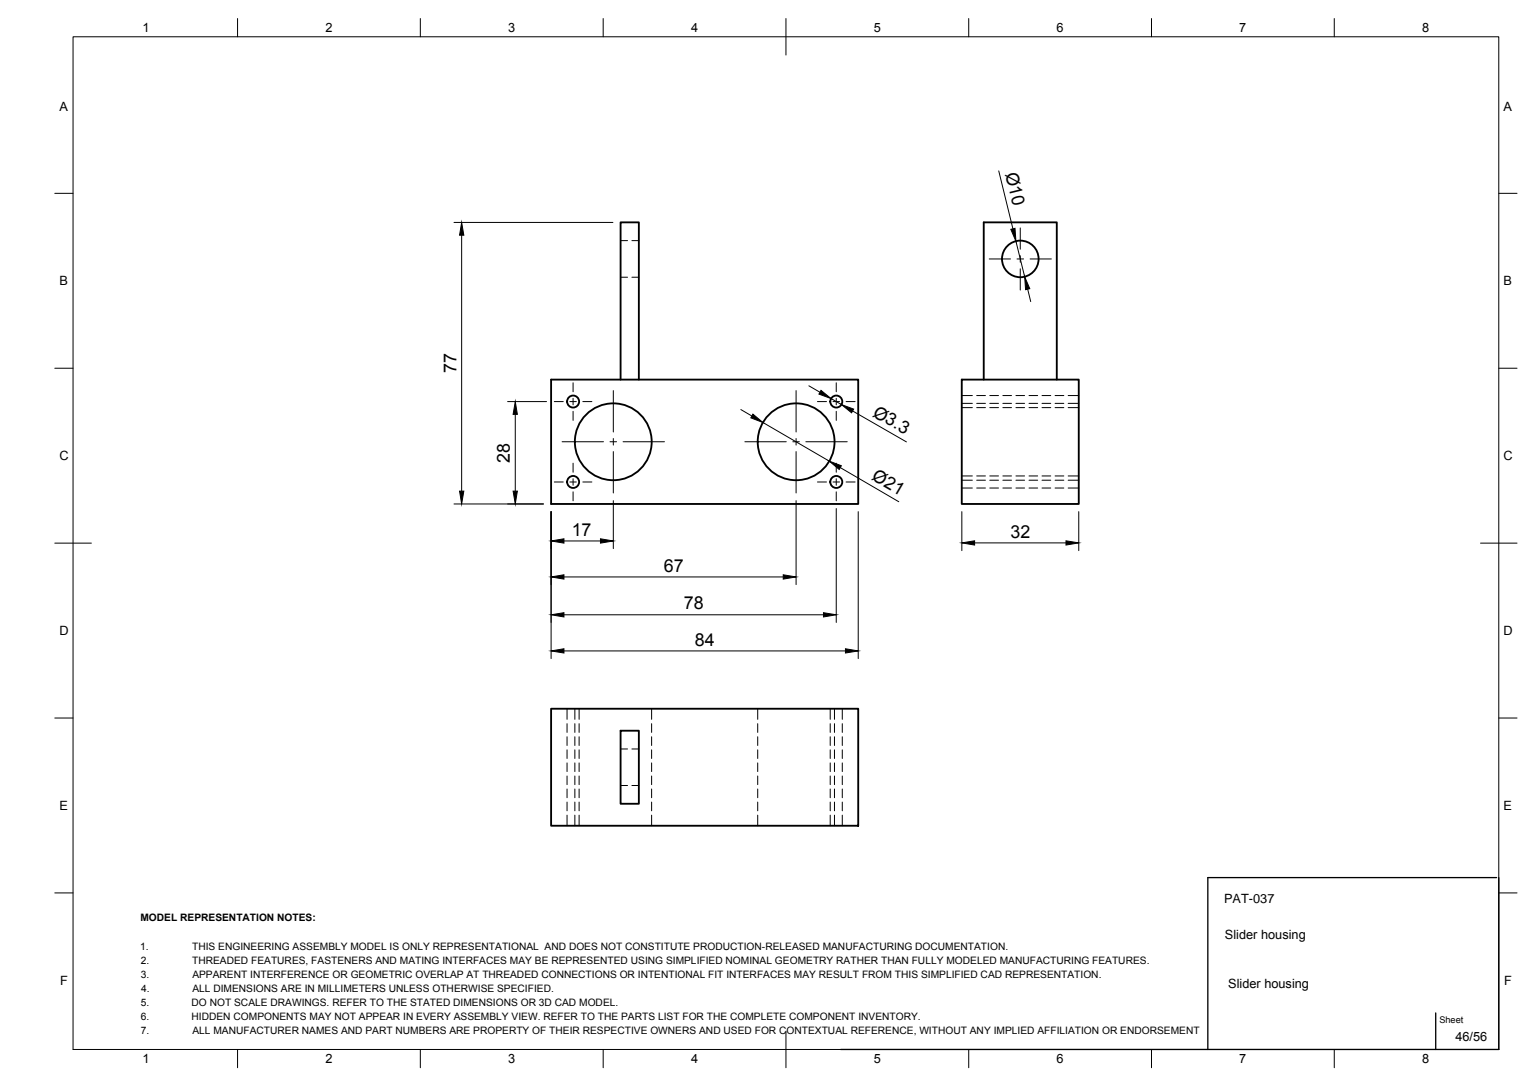
ISO-10303-21;
HEADER;
/* Generated by software containing ST-Developer
 * from STEP Tools, Inc. (www.steptools.com) 
 */

FILE_DESCRIPTION(
/* description */ ('Flywheel Crank-Slider'),
/* implementation_level */ '2;1');

FILE_NAME(
/* name */ 'Slider housing.step',
/* time_stamp */ '2026-10-28T03:23:13-07:00',
/* author */ (''),
/* organization */ (''),
/* preprocessor_version */ 'ST-DEVELOPER v20.2',
/* originating_system */ 'Autodesk Translation Framework v15.17.0.0',
/* authorisation */ '');

FILE_SCHEMA (('AUTOMOTIVE_DESIGN { 1 0 10303 214 3 1 1 }'));
ENDSEC;

DATA;
#10=MECHANICAL_DESIGN_GEOMETRIC_PRESENTATION_REPRESENTATION('',(#719),#17322);
#606=SHAPE_REPRESENTATION_RELATIONSHIP('SRR','None',#17607,#658);
#658=ADVANCED_BREP_SHAPE_REPRESENTATION('',(#776),#17311);
#719=STYLED_ITEM('',(#17910),#776);
#776=MANIFOLD_SOLID_BREP('Body1',#9101);
#952=FACE_BOUND('',#2457,.T.);
#953=FACE_BOUND('',#2462,.T.);
#954=FACE_BOUND('',#2471,.T.);
#955=FACE_BOUND('',#2472,.T.);
#956=FACE_BOUND('',#2473,.T.);
#957=FACE_BOUND('',#2474,.T.);
#958=FACE_BOUND('',#2475,.T.);
#959=FACE_BOUND('',#2476,.T.);
#960=FACE_BOUND('',#2479,.T.);
#961=FACE_BOUND('',#2480,.T.);
#962=FACE_BOUND('',#2481,.T.);
#963=FACE_BOUND('',#2482,.T.);
#964=FACE_BOUND('',#2483,.T.);
#965=FACE_BOUND('',#2484,.T.);
#966=FACE_BOUND('',#2486,.T.);
#1259=PLANE('',#10539);
#1260=PLANE('',#10540);
#1261=PLANE('',#10541);
#1262=PLANE('',#10542);
#1263=PLANE('',#10543);
#1264=PLANE('',#10562);
#1265=PLANE('',#10563);
#1266=PLANE('',#10564);
#1267=PLANE('',#10565);
#1268=PLANE('',#10566);
#1269=PLANE('',#10567);
#1753=FACE_OUTER_BOUND('',#2455,.T.);
#1754=FACE_OUTER_BOUND('',#2456,.T.);
#1755=FACE_OUTER_BOUND('',#2458,.T.);
#1756=FACE_OUTER_BOUND('',#2459,.T.);
#1757=FACE_OUTER_BOUND('',#2460,.T.);
#1758=FACE_OUTER_BOUND('',#2461,.T.);
#1759=FACE_OUTER_BOUND('',#2463,.T.);
#1760=FACE_OUTER_BOUND('',#2464,.T.);
#1761=FACE_OUTER_BOUND('',#2465,.T.);
#1762=FACE_OUTER_BOUND('',#2466,.T.);
#1763=FACE_OUTER_BOUND('',#2467,.T.);
#1764=FACE_OUTER_BOUND('',#2468,.T.);
#1765=FACE_OUTER_BOUND('',#2469,.T.);
#1766=FACE_OUTER_BOUND('',#2470,.T.);
#1767=FACE_OUTER_BOUND('',#2477,.T.);
#1768=FACE_OUTER_BOUND('',#2478,.T.);
#1769=FACE_OUTER_BOUND('',#2485,.T.);
#1770=FACE_OUTER_BOUND('',#2487,.T.);
#2455=EDGE_LOOP('',(#7910,#7911,#7912,#7913));
#2456=EDGE_LOOP('',(#7914,#7915,#7916,#7917));
#2457=EDGE_LOOP('',(#7918));
#2458=EDGE_LOOP('',(#7919,#7920,#7921,#7922));
#2459=EDGE_LOOP('',(#7923,#7924,#7925,#7926));
#2460=EDGE_LOOP('',(#7927,#7928,#7929,#7930));
#2461=EDGE_LOOP('',(#7931,#7932,#7933,#7934));
#2462=EDGE_LOOP('',(#7935));
#2463=EDGE_LOOP('',(#7936,#7937,#7938,#7939));
#2464=EDGE_LOOP('',(#7940,#7941,#7942,#7943));
#2465=EDGE_LOOP('',(#7944,#7945,#7946,#7947));
#2466=EDGE_LOOP('',(#7948,#7949,#7950,#7951));
#2467=EDGE_LOOP('',(#7952,#7953,#7954,#7955));
#2468=EDGE_LOOP('',(#7956,#7957,#7958,#7959));
#2469=EDGE_LOOP('',(#7960,#7961,#7962,#7963));
#2470=EDGE_LOOP('',(#7964,#7965,#7966,#7967));
#2471=EDGE_LOOP('',(#7968));
#2472=EDGE_LOOP('',(#7969));
#2473=EDGE_LOOP('',(#7970));
#2474=EDGE_LOOP('',(#7971));
#2475=EDGE_LOOP('',(#7972));
#2476=EDGE_LOOP('',(#7973));
#2477=EDGE_LOOP('',(#7974,#7975,#7976,#7977));
#2478=EDGE_LOOP('',(#7978,#7979,#7980,#7981));
#2479=EDGE_LOOP('',(#7982));
#2480=EDGE_LOOP('',(#7983));
#2481=EDGE_LOOP('',(#7984));
#2482=EDGE_LOOP('',(#7985));
#2483=EDGE_LOOP('',(#7986));
#2484=EDGE_LOOP('',(#7987));
#2485=EDGE_LOOP('',(#7988,#7989,#7990,#7991));
#2486=EDGE_LOOP('',(#7992,#7993,#7994,#7995));
#2487=EDGE_LOOP('',(#7996,#7997,#7998,#7999));
#3102=LINE('',#16647,#3713);
#3103=LINE('',#16652,#3714);
#3104=LINE('',#16654,#3715);
#3105=LINE('',#16656,#3716);
#3106=LINE('',#16657,#3717);
#3107=LINE('',#16660,#3718);
#3108=LINE('',#16662,#3719);
#3109=LINE('',#16663,#3720);
#3110=LINE('',#16666,#3721);
#3111=LINE('',#16668,#3722);
#3112=LINE('',#16669,#3723);
#3113=LINE('',#16671,#3724);
#3114=LINE('',#16673,#3725);
#3115=LINE('',#16678,#3726);
#3116=LINE('',#16684,#3727);
#3117=LINE('',#16690,#3728);
#3118=LINE('',#16696,#3729);
#3119=LINE('',#16702,#3730);
#3120=LINE('',#16708,#3731);
#3121=LINE('',#16713,#3732);
#3122=LINE('',#16715,#3733);
#3123=LINE('',#16717,#3734);
#3124=LINE('',#16718,#3735);
#3125=LINE('',#16721,#3736);
#3126=LINE('',#16723,#3737);
#3127=LINE('',#16724,#3738);
#3128=LINE('',#16727,#3739);
#3129=LINE('',#16729,#3740);
#3130=LINE('',#16730,#3741);
#3131=LINE('',#16732,#3742);
#3132=LINE('',#16733,#3743);
#3713=VECTOR('',#13022,0.5);
#3714=VECTOR('',#13027,1.);
#3715=VECTOR('',#13028,1.);
#3716=VECTOR('',#13029,1.);
#3717=VECTOR('',#13030,1.);
#3718=VECTOR('',#13033,1.);
#3719=VECTOR('',#13034,1.);
#3720=VECTOR('',#13035,1.);
#3721=VECTOR('',#13038,1.);
#3722=VECTOR('',#13039,1.);
#3723=VECTOR('',#13040,1.);
#3724=VECTOR('',#13043,1.);
#3725=VECTOR('',#13046,1.);
#3726=VECTOR('',#13051,0.165);
#3727=VECTOR('',#13058,0.165);
#3728=VECTOR('',#13065,0.165);
#3729=VECTOR('',#13072,0.165);
#3730=VECTOR('',#13079,1.05);
#3731=VECTOR('',#13086,1.05);
#3732=VECTOR('',#13091,1.);
#3733=VECTOR('',#13092,1.);
#3734=VECTOR('',#13093,1.);
#3735=VECTOR('',#13094,1.);
#3736=VECTOR('',#13097,1.);
#3737=VECTOR('',#13098,1.);
#3738=VECTOR('',#13099,1.);
#3739=VECTOR('',#13102,1.);
#3740=VECTOR('',#13103,1.);
#3741=VECTOR('',#13104,1.);
#3742=VECTOR('',#13107,1.);
#3743=VECTOR('',#13108,1.);
#4192=CIRCLE('',#10537,0.5);
#4193=CIRCLE('',#10538,0.5);
#4194=CIRCLE('',#10545,0.165);
#4195=CIRCLE('',#10546,0.165);
#4196=CIRCLE('',#10548,0.165);
#4197=CIRCLE('',#10549,0.165);
#4198=CIRCLE('',#10551,0.165);
#4199=CIRCLE('',#10552,0.165);
#4200=CIRCLE('',#10554,0.165);
#4201=CIRCLE('',#10555,0.165);
#4202=CIRCLE('',#10557,1.05);
#4203=CIRCLE('',#10558,1.05);
#4204=CIRCLE('',#10560,1.05);
#4205=CIRCLE('',#10561,1.05);
#4879=VERTEX_POINT('',#16644);
#4880=VERTEX_POINT('',#16646);
#4881=VERTEX_POINT('',#16650);
#4882=VERTEX_POINT('',#16651);
#4883=VERTEX_POINT('',#16653);
#4884=VERTEX_POINT('',#16655);
#4885=VERTEX_POINT('',#16659);
#4886=VERTEX_POINT('',#16661);
#4887=VERTEX_POINT('',#16665);
#4888=VERTEX_POINT('',#16667);
#4889=VERTEX_POINT('',#16675);
#4890=VERTEX_POINT('',#16677);
#4891=VERTEX_POINT('',#16681);
#4892=VERTEX_POINT('',#16683);
#4893=VERTEX_POINT('',#16687);
#4894=VERTEX_POINT('',#16689);
#4895=VERTEX_POINT('',#16693);
#4896=VERTEX_POINT('',#16695);
#4897=VERTEX_POINT('',#16699);
#4898=VERTEX_POINT('',#16701);
#4899=VERTEX_POINT('',#16705);
#4900=VERTEX_POINT('',#16707);
#4901=VERTEX_POINT('',#16711);
#4902=VERTEX_POINT('',#16712);
#4903=VERTEX_POINT('',#16714);
#4904=VERTEX_POINT('',#16716);
#4905=VERTEX_POINT('',#16720);
#4906=VERTEX_POINT('',#16722);
#4907=VERTEX_POINT('',#16726);
#4908=VERTEX_POINT('',#16728);
#5912=EDGE_CURVE('',#4879,#4879,#4192,.T.);
#5913=EDGE_CURVE('',#4879,#4880,#3102,.T.);
#5914=EDGE_CURVE('',#4880,#4880,#4193,.T.);
#5915=EDGE_CURVE('',#4881,#4882,#3103,.T.);
#5916=EDGE_CURVE('',#4881,#4883,#3104,.T.);
#5917=EDGE_CURVE('',#4883,#4884,#3105,.T.);
#5918=EDGE_CURVE('',#4884,#4882,#3106,.T.);
#5919=EDGE_CURVE('',#4885,#4881,#3107,.T.);
#5920=EDGE_CURVE('',#4886,#4885,#3108,.T.);
#5921=EDGE_CURVE('',#4883,#4886,#3109,.T.);
#5922=EDGE_CURVE('',#4882,#4887,#3110,.T.);
#5923=EDGE_CURVE('',#4884,#4888,#3111,.T.);
#5924=EDGE_CURVE('',#4887,#4888,#3112,.T.);
#5925=EDGE_CURVE('',#4888,#4886,#3113,.T.);
#5926=EDGE_CURVE('',#4887,#4885,#3114,.T.);
#5927=EDGE_CURVE('',#4889,#4889,#4194,.T.);
#5928=EDGE_CURVE('',#4889,#4890,#3115,.T.);
#5929=EDGE_CURVE('',#4890,#4890,#4195,.T.);
#5930=EDGE_CURVE('',#4891,#4891,#4196,.T.);
#5931=EDGE_CURVE('',#4891,#4892,#3116,.T.);
#5932=EDGE_CURVE('',#4892,#4892,#4197,.T.);
#5933=EDGE_CURVE('',#4893,#4893,#4198,.T.);
#5934=EDGE_CURVE('',#4893,#4894,#3117,.T.);
#5935=EDGE_CURVE('',#4894,#4894,#4199,.T.);
#5936=EDGE_CURVE('',#4895,#4895,#4200,.T.);
#5937=EDGE_CURVE('',#4895,#4896,#3118,.T.);
#5938=EDGE_CURVE('',#4896,#4896,#4201,.T.);
#5939=EDGE_CURVE('',#4897,#4897,#4202,.T.);
#5940=EDGE_CURVE('',#4897,#4898,#3119,.T.);
#5941=EDGE_CURVE('',#4898,#4898,#4203,.T.);
#5942=EDGE_CURVE('',#4899,#4899,#4204,.T.);
#5943=EDGE_CURVE('',#4899,#4900,#3120,.T.);
#5944=EDGE_CURVE('',#4900,#4900,#4205,.T.);
#5945=EDGE_CURVE('',#4901,#4902,#3121,.T.);
#5946=EDGE_CURVE('',#4902,#4903,#3122,.T.);
#5947=EDGE_CURVE('',#4904,#4903,#3123,.T.);
#5948=EDGE_CURVE('',#4901,#4904,#3124,.T.);
#5949=EDGE_CURVE('',#4905,#4901,#3125,.T.);
#5950=EDGE_CURVE('',#4906,#4904,#3126,.T.);
#5951=EDGE_CURVE('',#4905,#4906,#3127,.T.);
#5952=EDGE_CURVE('',#4907,#4905,#3128,.T.);
#5953=EDGE_CURVE('',#4908,#4906,#3129,.T.);
#5954=EDGE_CURVE('',#4907,#4908,#3130,.T.);
#5955=EDGE_CURVE('',#4902,#4907,#3131,.T.);
#5956=EDGE_CURVE('',#4903,#4908,#3132,.T.);
#7910=ORIENTED_EDGE('',*,*,#5912,.F.);
#7911=ORIENTED_EDGE('',*,*,#5913,.T.);
#7912=ORIENTED_EDGE('',*,*,#5914,.F.);
#7913=ORIENTED_EDGE('',*,*,#5913,.F.);
#7914=ORIENTED_EDGE('',*,*,#5915,.F.);
#7915=ORIENTED_EDGE('',*,*,#5916,.T.);
#7916=ORIENTED_EDGE('',*,*,#5917,.T.);
#7917=ORIENTED_EDGE('',*,*,#5918,.T.);
#7918=ORIENTED_EDGE('',*,*,#5912,.T.);
#7919=ORIENTED_EDGE('',*,*,#5919,.F.);
#7920=ORIENTED_EDGE('',*,*,#5920,.F.);
#7921=ORIENTED_EDGE('',*,*,#5921,.F.);
#7922=ORIENTED_EDGE('',*,*,#5916,.F.);
#7923=ORIENTED_EDGE('',*,*,#5922,.F.);
#7924=ORIENTED_EDGE('',*,*,#5918,.F.);
#7925=ORIENTED_EDGE('',*,*,#5923,.T.);
#7926=ORIENTED_EDGE('',*,*,#5924,.F.);
#7927=ORIENTED_EDGE('',*,*,#5917,.F.);
#7928=ORIENTED_EDGE('',*,*,#5921,.T.);
#7929=ORIENTED_EDGE('',*,*,#5925,.F.);
#7930=ORIENTED_EDGE('',*,*,#5923,.F.);
#7931=ORIENTED_EDGE('',*,*,#5926,.F.);
#7932=ORIENTED_EDGE('',*,*,#5924,.T.);
#7933=ORIENTED_EDGE('',*,*,#5925,.T.);
#7934=ORIENTED_EDGE('',*,*,#5920,.T.);
#7935=ORIENTED_EDGE('',*,*,#5914,.T.);
#7936=ORIENTED_EDGE('',*,*,#5927,.F.);
#7937=ORIENTED_EDGE('',*,*,#5928,.T.);
#7938=ORIENTED_EDGE('',*,*,#5929,.F.);
#7939=ORIENTED_EDGE('',*,*,#5928,.F.);
#7940=ORIENTED_EDGE('',*,*,#5930,.F.);
#7941=ORIENTED_EDGE('',*,*,#5931,.T.);
#7942=ORIENTED_EDGE('',*,*,#5932,.F.);
#7943=ORIENTED_EDGE('',*,*,#5931,.F.);
#7944=ORIENTED_EDGE('',*,*,#5933,.F.);
#7945=ORIENTED_EDGE('',*,*,#5934,.T.);
#7946=ORIENTED_EDGE('',*,*,#5935,.F.);
#7947=ORIENTED_EDGE('',*,*,#5934,.F.);
#7948=ORIENTED_EDGE('',*,*,#5936,.F.);
#7949=ORIENTED_EDGE('',*,*,#5937,.T.);
#7950=ORIENTED_EDGE('',*,*,#5938,.F.);
#7951=ORIENTED_EDGE('',*,*,#5937,.F.);
#7952=ORIENTED_EDGE('',*,*,#5939,.F.);
#7953=ORIENTED_EDGE('',*,*,#5940,.T.);
#7954=ORIENTED_EDGE('',*,*,#5941,.F.);
#7955=ORIENTED_EDGE('',*,*,#5940,.F.);
#7956=ORIENTED_EDGE('',*,*,#5942,.F.);
#7957=ORIENTED_EDGE('',*,*,#5943,.T.);
#7958=ORIENTED_EDGE('',*,*,#5944,.F.);
#7959=ORIENTED_EDGE('',*,*,#5943,.F.);
#7960=ORIENTED_EDGE('',*,*,#5945,.T.);
#7961=ORIENTED_EDGE('',*,*,#5946,.T.);
#7962=ORIENTED_EDGE('',*,*,#5947,.F.);
#7963=ORIENTED_EDGE('',*,*,#5948,.F.);
#7964=ORIENTED_EDGE('',*,*,#5949,.T.);
#7965=ORIENTED_EDGE('',*,*,#5948,.T.);
#7966=ORIENTED_EDGE('',*,*,#5950,.F.);
#7967=ORIENTED_EDGE('',*,*,#5951,.F.);
#7968=ORIENTED_EDGE('',*,*,#5944,.T.);
#7969=ORIENTED_EDGE('',*,*,#5941,.T.);
#7970=ORIENTED_EDGE('',*,*,#5938,.T.);
#7971=ORIENTED_EDGE('',*,*,#5935,.T.);
#7972=ORIENTED_EDGE('',*,*,#5932,.T.);
#7973=ORIENTED_EDGE('',*,*,#5929,.T.);
#7974=ORIENTED_EDGE('',*,*,#5952,.T.);
#7975=ORIENTED_EDGE('',*,*,#5951,.T.);
#7976=ORIENTED_EDGE('',*,*,#5953,.F.);
#7977=ORIENTED_EDGE('',*,*,#5954,.F.);
#7978=ORIENTED_EDGE('',*,*,#5955,.T.);
#7979=ORIENTED_EDGE('',*,*,#5954,.T.);
#7980=ORIENTED_EDGE('',*,*,#5956,.F.);
#7981=ORIENTED_EDGE('',*,*,#5946,.F.);
#7982=ORIENTED_EDGE('',*,*,#5942,.T.);
#7983=ORIENTED_EDGE('',*,*,#5939,.T.);
#7984=ORIENTED_EDGE('',*,*,#5936,.T.);
#7985=ORIENTED_EDGE('',*,*,#5933,.T.);
#7986=ORIENTED_EDGE('',*,*,#5930,.T.);
#7987=ORIENTED_EDGE('',*,*,#5927,.T.);
#7988=ORIENTED_EDGE('',*,*,#5956,.T.);
#7989=ORIENTED_EDGE('',*,*,#5953,.T.);
#7990=ORIENTED_EDGE('',*,*,#5950,.T.);
#7991=ORIENTED_EDGE('',*,*,#5947,.T.);
#7992=ORIENTED_EDGE('',*,*,#5919,.T.);
#7993=ORIENTED_EDGE('',*,*,#5915,.T.);
#7994=ORIENTED_EDGE('',*,*,#5922,.T.);
#7995=ORIENTED_EDGE('',*,*,#5926,.T.);
#7996=ORIENTED_EDGE('',*,*,#5955,.F.);
#7997=ORIENTED_EDGE('',*,*,#5945,.F.);
#7998=ORIENTED_EDGE('',*,*,#5949,.F.);
#7999=ORIENTED_EDGE('',*,*,#5952,.F.);
#8473=CYLINDRICAL_SURFACE('',#10536,0.5);
#8474=CYLINDRICAL_SURFACE('',#10544,0.165);
#8475=CYLINDRICAL_SURFACE('',#10547,0.165);
#8476=CYLINDRICAL_SURFACE('',#10550,0.165);
#8477=CYLINDRICAL_SURFACE('',#10553,0.165);
#8478=CYLINDRICAL_SURFACE('',#10556,1.05);
#8479=CYLINDRICAL_SURFACE('',#10559,1.05);
#8944=ADVANCED_FACE('',(#1753),#8473,.F.);
#8945=ADVANCED_FACE('',(#1754,#952),#1259,.F.);
#8946=ADVANCED_FACE('',(#1755),#1260,.T.);
#8947=ADVANCED_FACE('',(#1756),#1261,.T.);
#8948=ADVANCED_FACE('',(#1757),#1262,.T.);
#8949=ADVANCED_FACE('',(#1758,#953),#1263,.T.);
#8950=ADVANCED_FACE('',(#1759),#8474,.F.);
#8951=ADVANCED_FACE('',(#1760),#8475,.F.);
#8952=ADVANCED_FACE('',(#1761),#8476,.F.);
#8953=ADVANCED_FACE('',(#1762),#8477,.F.);
#8954=ADVANCED_FACE('',(#1763),#8478,.F.);
#8955=ADVANCED_FACE('',(#1764),#8479,.F.);
#8956=ADVANCED_FACE('',(#1765),#1264,.T.);
#8957=ADVANCED_FACE('',(#1766,#954,#955,#956,#957,#958,#959),#1265,.T.);
#8958=ADVANCED_FACE('',(#1767),#1266,.T.);
#8959=ADVANCED_FACE('',(#1768,#960,#961,#962,#963,#964,#965),#1267,.T.);
#8960=ADVANCED_FACE('',(#1769,#966),#1268,.T.);
#8961=ADVANCED_FACE('',(#1770),#1269,.F.);
#9101=CLOSED_SHELL('',(#8944,#8945,#8946,#8947,#8948,#8949,#8950,#8951,
#8952,#8953,#8954,#8955,#8956,#8957,#8958,#8959,#8960,#8961));
#10535=AXIS2_PLACEMENT_3D('',#16642,#13016,#13017);
#10536=AXIS2_PLACEMENT_3D('',#16643,#13018,#13019);
#10537=AXIS2_PLACEMENT_3D('',#16645,#13020,#13021);
#10538=AXIS2_PLACEMENT_3D('',#16648,#13023,#13024);
#10539=AXIS2_PLACEMENT_3D('',#16649,#13025,#13026);
#10540=AXIS2_PLACEMENT_3D('',#16658,#13031,#13032);
#10541=AXIS2_PLACEMENT_3D('',#16664,#13036,#13037);
#10542=AXIS2_PLACEMENT_3D('',#16670,#13041,#13042);
#10543=AXIS2_PLACEMENT_3D('',#16672,#13044,#13045);
#10544=AXIS2_PLACEMENT_3D('',#16674,#13047,#13048);
#10545=AXIS2_PLACEMENT_3D('',#16676,#13049,#13050);
#10546=AXIS2_PLACEMENT_3D('',#16679,#13052,#13053);
#10547=AXIS2_PLACEMENT_3D('',#16680,#13054,#13055);
#10548=AXIS2_PLACEMENT_3D('',#16682,#13056,#13057);
#10549=AXIS2_PLACEMENT_3D('',#16685,#13059,#13060);
#10550=AXIS2_PLACEMENT_3D('',#16686,#13061,#13062);
#10551=AXIS2_PLACEMENT_3D('',#16688,#13063,#13064);
#10552=AXIS2_PLACEMENT_3D('',#16691,#13066,#13067);
#10553=AXIS2_PLACEMENT_3D('',#16692,#13068,#13069);
#10554=AXIS2_PLACEMENT_3D('',#16694,#13070,#13071);
#10555=AXIS2_PLACEMENT_3D('',#16697,#13073,#13074);
#10556=AXIS2_PLACEMENT_3D('',#16698,#13075,#13076);
#10557=AXIS2_PLACEMENT_3D('',#16700,#13077,#13078);
#10558=AXIS2_PLACEMENT_3D('',#16703,#13080,#13081);
#10559=AXIS2_PLACEMENT_3D('',#16704,#13082,#13083);
#10560=AXIS2_PLACEMENT_3D('',#16706,#13084,#13085);
#10561=AXIS2_PLACEMENT_3D('',#16709,#13087,#13088);
#10562=AXIS2_PLACEMENT_3D('',#16710,#13089,#13090);
#10563=AXIS2_PLACEMENT_3D('',#16719,#13095,#13096);
#10564=AXIS2_PLACEMENT_3D('',#16725,#13100,#13101);
#10565=AXIS2_PLACEMENT_3D('',#16731,#13105,#13106);
#10566=AXIS2_PLACEMENT_3D('',#16734,#13109,#13110);
#10567=AXIS2_PLACEMENT_3D('',#16735,#13111,#13112);
#13016=DIRECTION('axis',(0.,0.,1.));
#13017=DIRECTION('refdir',(1.,0.,0.));
#13018=DIRECTION('center_axis',(0.,1.,0.));
#13019=DIRECTION('ref_axis',(1.,0.,0.));
#13020=DIRECTION('center_axis',(0.,1.,0.));
#13021=DIRECTION('ref_axis',(1.,0.,0.));
#13022=DIRECTION('',(0.,1.,0.));
#13023=DIRECTION('center_axis',(0.,-1.,0.));
#13024=DIRECTION('ref_axis',(1.,0.,0.));
#13025=DIRECTION('center_axis',(0.,1.,0.));
#13026=DIRECTION('ref_axis',(1.,0.,0.));
#13027=DIRECTION('',(-1.,0.,0.));
#13028=DIRECTION('',(0.,0.,1.));
#13029=DIRECTION('',(-1.,0.,0.));
#13030=DIRECTION('',(0.,0.,-1.));
#13031=DIRECTION('center_axis',(1.,0.,0.));
#13032=DIRECTION('ref_axis',(0.,0.,-1.));
#13033=DIRECTION('',(0.,-1.,0.));
#13034=DIRECTION('',(0.,0.,-1.));
#13035=DIRECTION('',(0.,1.,0.));
#13036=DIRECTION('center_axis',(-1.,0.,0.));
#13037=DIRECTION('ref_axis',(0.,0.,1.));
#13038=DIRECTION('',(0.,1.,0.));
#13039=DIRECTION('',(0.,1.,0.));
#13040=DIRECTION('',(0.,0.,1.));
#13041=DIRECTION('center_axis',(0.,0.,1.));
#13042=DIRECTION('ref_axis',(1.,0.,0.));
#13043=DIRECTION('',(1.,0.,0.));
#13044=DIRECTION('center_axis',(0.,1.,0.));
#13045=DIRECTION('ref_axis',(0.,0.,1.));
#13046=DIRECTION('',(1.,0.,0.));
#13047=DIRECTION('center_axis',(1.,0.,0.));
#13048=DIRECTION('ref_axis',(0.,0.,-1.));
#13049=DIRECTION('center_axis',(1.,0.,0.));
#13050=DIRECTION('ref_axis',(0.,0.,-1.));
#13051=DIRECTION('',(1.,0.,0.));
#13052=DIRECTION('center_axis',(-1.,0.,0.));
#13053=DIRECTION('ref_axis',(0.,0.,-1.));
#13054=DIRECTION('center_axis',(1.,0.,0.));
#13055=DIRECTION('ref_axis',(0.,0.,-1.));
#13056=DIRECTION('center_axis',(1.,0.,0.));
#13057=DIRECTION('ref_axis',(0.,0.,-1.));
#13058=DIRECTION('',(1.,0.,0.));
#13059=DIRECTION('center_axis',(-1.,0.,0.));
#13060=DIRECTION('ref_axis',(0.,0.,-1.));
#13061=DIRECTION('center_axis',(1.,0.,0.));
#13062=DIRECTION('ref_axis',(0.,0.,-1.));
#13063=DIRECTION('center_axis',(1.,0.,0.));
#13064=DIRECTION('ref_axis',(0.,0.,-1.));
#13065=DIRECTION('',(1.,0.,0.));
#13066=DIRECTION('center_axis',(-1.,0.,0.));
#13067=DIRECTION('ref_axis',(0.,0.,-1.));
#13068=DIRECTION('center_axis',(1.,0.,0.));
#13069=DIRECTION('ref_axis',(0.,0.,-1.));
#13070=DIRECTION('center_axis',(1.,0.,0.));
#13071=DIRECTION('ref_axis',(0.,0.,-1.));
#13072=DIRECTION('',(1.,0.,0.));
#13073=DIRECTION('center_axis',(-1.,0.,0.));
#13074=DIRECTION('ref_axis',(0.,0.,-1.));
#13075=DIRECTION('center_axis',(1.,0.,0.));
#13076=DIRECTION('ref_axis',(0.,0.,-1.));
#13077=DIRECTION('center_axis',(1.,0.,0.));
#13078=DIRECTION('ref_axis',(0.,0.,-1.));
#13079=DIRECTION('',(1.,0.,0.));
#13080=DIRECTION('center_axis',(-1.,0.,0.));
#13081=DIRECTION('ref_axis',(0.,0.,-1.));
#13082=DIRECTION('center_axis',(1.,0.,0.));
#13083=DIRECTION('ref_axis',(0.,0.,-1.));
#13084=DIRECTION('center_axis',(1.,0.,0.));
#13085=DIRECTION('ref_axis',(0.,0.,-1.));
#13086=DIRECTION('',(1.,0.,0.));
#13087=DIRECTION('center_axis',(-1.,0.,0.));
#13088=DIRECTION('ref_axis',(0.,0.,-1.));
#13089=DIRECTION('center_axis',(0.,1.,0.));
#13090=DIRECTION('ref_axis',(-1.,0.,0.));
#13091=DIRECTION('',(-1.,0.,0.));
#13092=DIRECTION('',(0.,0.,1.));
#13093=DIRECTION('',(-1.,0.,0.));
#13094=DIRECTION('',(0.,0.,1.));
#13095=DIRECTION('center_axis',(1.,0.,0.));
#13096=DIRECTION('ref_axis',(0.,1.,0.));
#13097=DIRECTION('',(0.,1.,0.));
#13098=DIRECTION('',(0.,1.,0.));
#13099=DIRECTION('',(0.,0.,1.));
#13100=DIRECTION('center_axis',(0.,-1.,0.));
#13101=DIRECTION('ref_axis',(1.,0.,0.));
#13102=DIRECTION('',(1.,0.,0.));
#13103=DIRECTION('',(1.,0.,0.));
#13104=DIRECTION('',(0.,0.,1.));
#13105=DIRECTION('center_axis',(-1.,0.,0.));
#13106=DIRECTION('ref_axis',(0.,-1.,0.));
#13107=DIRECTION('',(0.,-1.,0.));
#13108=DIRECTION('',(0.,-1.,0.));
#13109=DIRECTION('center_axis',(0.,0.,1.));
#13110=DIRECTION('ref_axis',(1.,0.,0.));
#13111=DIRECTION('center_axis',(0.,0.,1.));
#13112=DIRECTION('ref_axis',(1.,0.,0.));
#16642=CARTESIAN_POINT('',(0.,0.,0.));
#16643=CARTESIAN_POINT('Origin',(12.,1.7,10.));
#16644=CARTESIAN_POINT('',(11.5,1.8,10.));
#16645=CARTESIAN_POINT('Origin',(12.,1.8,10.));
#16646=CARTESIAN_POINT('',(11.5,2.3,10.));
#16647=CARTESIAN_POINT('',(11.5,1.7,10.));
#16648=CARTESIAN_POINT('Origin',(12.,2.3,10.));
#16649=CARTESIAN_POINT('Origin',(12.,1.8,8.75));
#16650=CARTESIAN_POINT('',(13.,1.8,6.7));
#16651=CARTESIAN_POINT('',(11.,1.8,6.7));
#16652=CARTESIAN_POINT('',(12.,1.8,6.7));
#16653=CARTESIAN_POINT('',(13.,1.8,11.));
#16654=CARTESIAN_POINT('',(13.,1.8,6.5));
#16655=CARTESIAN_POINT('',(11.,1.8,11.));
#16656=CARTESIAN_POINT('',(13.,1.8,11.));
#16657=CARTESIAN_POINT('',(11.,1.8,11.));
#16658=CARTESIAN_POINT('Origin',(13.,1.8,11.));
#16659=CARTESIAN_POINT('',(13.,2.3,6.7));
#16660=CARTESIAN_POINT('',(13.,0.9,6.7));
#16661=CARTESIAN_POINT('',(13.,2.3,11.));
#16662=CARTESIAN_POINT('',(13.,2.3,6.5));
#16663=CARTESIAN_POINT('',(13.,1.8,11.));
#16664=CARTESIAN_POINT('Origin',(11.,1.8,6.5));
#16665=CARTESIAN_POINT('',(11.,2.3,6.7));
#16666=CARTESIAN_POINT('',(11.,0.9,6.7));
#16667=CARTESIAN_POINT('',(11.,2.3,11.));
#16668=CARTESIAN_POINT('',(11.,1.8,11.));
#16669=CARTESIAN_POINT('',(11.,2.3,11.));
#16670=CARTESIAN_POINT('Origin',(11.,1.8,11.));
#16671=CARTESIAN_POINT('',(13.,2.3,11.));
#16672=CARTESIAN_POINT('Origin',(12.,2.3,8.75));
#16673=CARTESIAN_POINT('',(12.,2.3,6.7));
#16674=CARTESIAN_POINT('Origin',(10.3,3.6,3.9));
#16675=CARTESIAN_POINT('',(10.4,3.6,4.065));
#16676=CARTESIAN_POINT('Origin',(10.4,3.6,3.9));
#16677=CARTESIAN_POINT('',(13.6,3.6,4.065));
#16678=CARTESIAN_POINT('',(10.3,3.6,4.065));
#16679=CARTESIAN_POINT('Origin',(13.6,3.6,3.9));
#16680=CARTESIAN_POINT('Origin',(10.3,-3.6,6.1));
#16681=CARTESIAN_POINT('',(10.4,-3.6,6.265));
#16682=CARTESIAN_POINT('Origin',(10.4,-3.6,6.1));
#16683=CARTESIAN_POINT('',(13.6,-3.6,6.265));
#16684=CARTESIAN_POINT('',(10.3,-3.6,6.265));
#16685=CARTESIAN_POINT('Origin',(13.6,-3.6,6.1));
#16686=CARTESIAN_POINT('Origin',(10.3,-3.6,3.9));
#16687=CARTESIAN_POINT('',(10.4,-3.6,4.065));
#16688=CARTESIAN_POINT('Origin',(10.4,-3.6,3.9));
#16689=CARTESIAN_POINT('',(13.6,-3.6,4.065));
#16690=CARTESIAN_POINT('',(10.3,-3.6,4.065));
#16691=CARTESIAN_POINT('Origin',(13.6,-3.6,3.9));
#16692=CARTESIAN_POINT('Origin',(10.3,3.6,6.1));
#16693=CARTESIAN_POINT('',(10.4,3.6,6.265));
#16694=CARTESIAN_POINT('Origin',(10.4,3.6,6.1));
#16695=CARTESIAN_POINT('',(13.6,3.6,6.265));
#16696=CARTESIAN_POINT('',(10.3,3.6,6.265));
#16697=CARTESIAN_POINT('Origin',(13.6,3.6,6.1));
#16698=CARTESIAN_POINT('Origin',(10.3,-2.5,5.));
#16699=CARTESIAN_POINT('',(10.4,-2.5,6.05));
#16700=CARTESIAN_POINT('Origin',(10.4,-2.5,5.));
#16701=CARTESIAN_POINT('',(13.6,-2.5,6.05));
#16702=CARTESIAN_POINT('',(10.3,-2.5,6.05));
#16703=CARTESIAN_POINT('Origin',(13.6,-2.5,5.));
#16704=CARTESIAN_POINT('Origin',(10.3,2.5,5.));
#16705=CARTESIAN_POINT('',(10.4,2.5,6.05));
#16706=CARTESIAN_POINT('Origin',(10.4,2.5,5.));
#16707=CARTESIAN_POINT('',(13.6,2.5,6.05));
#16708=CARTESIAN_POINT('',(10.3,2.5,6.05));
#16709=CARTESIAN_POINT('Origin',(13.6,2.5,5.));
#16710=CARTESIAN_POINT('Origin',(13.6,4.2,3.3));
#16711=CARTESIAN_POINT('',(13.6,4.2,3.3));
#16712=CARTESIAN_POINT('',(10.4,4.2,3.3));
#16713=CARTESIAN_POINT('',(13.6,4.2,3.3));
#16714=CARTESIAN_POINT('',(10.4,4.2,6.7));
#16715=CARTESIAN_POINT('',(10.4,4.2,3.3));
#16716=CARTESIAN_POINT('',(13.6,4.2,6.7));
#16717=CARTESIAN_POINT('',(13.6,4.2,6.7));
#16718=CARTESIAN_POINT('',(13.6,4.2,3.3));
#16719=CARTESIAN_POINT('Origin',(13.6,-4.2,3.3));
#16720=CARTESIAN_POINT('',(13.6,-4.2,3.3));
#16721=CARTESIAN_POINT('',(13.6,-4.2,3.3));
#16722=CARTESIAN_POINT('',(13.6,-4.2,6.7));
#16723=CARTESIAN_POINT('',(13.6,-4.2,6.7));
#16724=CARTESIAN_POINT('',(13.6,-4.2,3.3));
#16725=CARTESIAN_POINT('Origin',(10.4,-4.2,3.3));
#16726=CARTESIAN_POINT('',(10.4,-4.2,3.3));
#16727=CARTESIAN_POINT('',(10.4,-4.2,3.3));
#16728=CARTESIAN_POINT('',(10.4,-4.2,6.7));
#16729=CARTESIAN_POINT('',(10.4,-4.2,6.7));
#16730=CARTESIAN_POINT('',(10.4,-4.2,3.3));
#16731=CARTESIAN_POINT('Origin',(10.4,4.2,3.3));
#16732=CARTESIAN_POINT('',(10.4,4.2,3.3));
#16733=CARTESIAN_POINT('',(10.4,4.2,6.7));
#16734=CARTESIAN_POINT('Origin',(12.,0.,6.7));
#16735=CARTESIAN_POINT('Origin',(12.,0.,3.3));
#17250=UNCERTAINTY_MEASURE_WITH_UNIT(LENGTH_MEASURE(0.001),#17323,
'DISTANCE_ACCURACY_VALUE',
'Maximum model space distance between geometric entities at asserted c
onnectivities');
#17261=UNCERTAINTY_MEASURE_WITH_UNIT(LENGTH_MEASURE(0.001),#17323,
'DISTANCE_ACCURACY_VALUE',
'Maximum model space distance between geometric entities at asserted c
onnectivities');
#17311=(
GEOMETRIC_REPRESENTATION_CONTEXT(3)
GLOBAL_UNCERTAINTY_ASSIGNED_CONTEXT((#17250))
GLOBAL_UNIT_ASSIGNED_CONTEXT((#17323,#17325,#17326))
REPRESENTATION_CONTEXT('','3D')
);
#17322=(
GEOMETRIC_REPRESENTATION_CONTEXT(3)
GLOBAL_UNCERTAINTY_ASSIGNED_CONTEXT((#17261))
GLOBAL_UNIT_ASSIGNED_CONTEXT((#17323,#17325,#17326))
REPRESENTATION_CONTEXT('','3D')
);
#17323=(
LENGTH_UNIT()
NAMED_UNIT(*)
SI_UNIT(.CENTI.,.METRE.)
);
#17325=(
NAMED_UNIT(*)
PLANE_ANGLE_UNIT()
SI_UNIT($,.RADIAN.)
);
#17326=(
NAMED_UNIT(*)
SI_UNIT($,.STERADIAN.)
SOLID_ANGLE_UNIT()
);
#17376=SHAPE_DEFINITION_REPRESENTATION(#17450,#17607);
#17450=PRODUCT_DEFINITION_SHAPE('',$,#17668);
#17607=SHAPE_REPRESENTATION('',(#10535),#17311);
#17618=PRODUCT_DEFINITION_CONTEXT('part definition',#17800,'design');
#17668=PRODUCT_DEFINITION('Slider housing','Slider housing',#17728,#17618);
#17728=PRODUCT_DEFINITION_FORMATION('',$,#17851);
#17800=APPLICATION_CONTEXT(
'Core Data for Automotive Mechanical Design Process');
#17801=PRODUCT_CONTEXT('part definition',#17800,'mechanical');
#17851=PRODUCT('Slider housing','Slider housing','Slider housing',(#17801));
#17904=COLOUR_RGB('Dark Blue',0.08,0.2,0.34);
#17905=FILL_AREA_STYLE_COLOUR('',#17904);
#17906=FILL_AREA_STYLE('',(#17905));
#17907=SURFACE_STYLE_FILL_AREA(#17906);
#17908=SURFACE_SIDE_STYLE('',(#17907));
#17909=SURFACE_STYLE_USAGE(.BOTH.,#17908);
#17910=PRESENTATION_STYLE_ASSIGNMENT((#17909));
ENDSEC;
END-ISO-10303-21;
